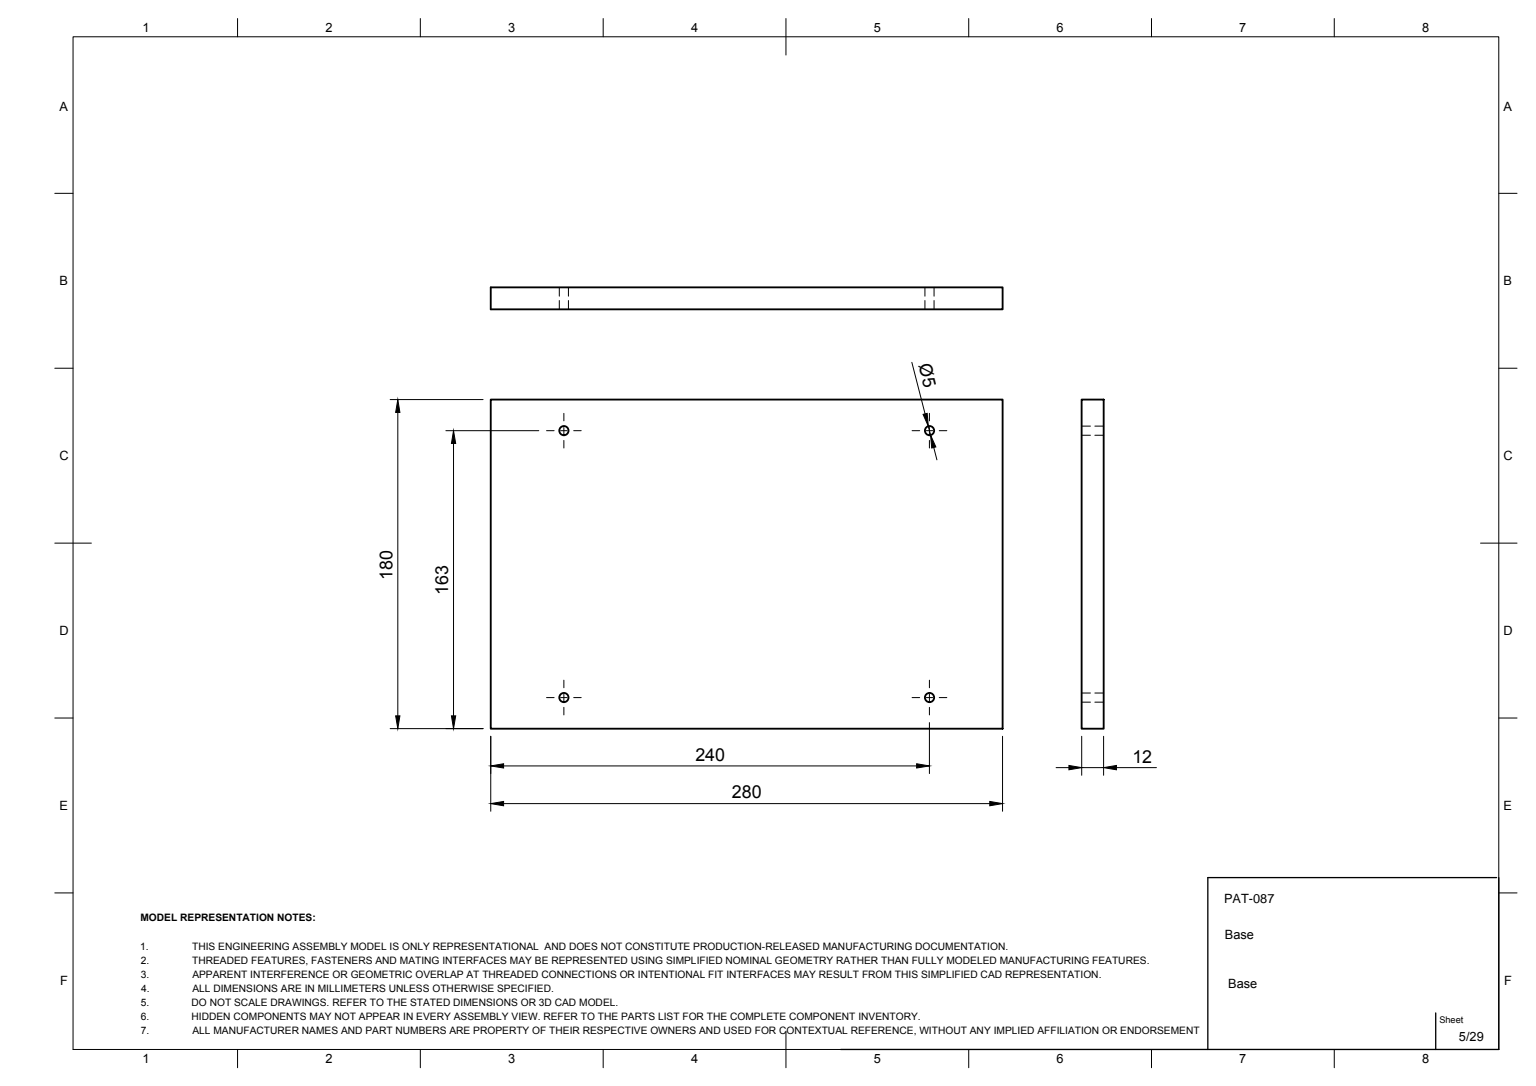
ISO-10303-21;
HEADER;
/* Generated by software containing ST-Developer
 * from STEP Tools, Inc. (www.steptools.com) 
 */

FILE_DESCRIPTION(
/* description */ ('Rigid flange shaft coupling assembly'),
/* implementation_level */ '2;1');

FILE_NAME(
/* name */ 'Base.step',
/* time_stamp */ '2026-10-27T10:47:16-07:00',
/* author */ (''),
/* organization */ (''),
/* preprocessor_version */ 'ST-DEVELOPER v20.2',
/* originating_system */ 'Autodesk Translation Framework v15.17.0.0',
/* authorisation */ '');

FILE_SCHEMA (('AUTOMOTIVE_DESIGN { 1 0 10303 214 3 1 1 }'));
ENDSEC;

DATA;
#10=MECHANICAL_DESIGN_GEOMETRIC_PRESENTATION_REPRESENTATION('',(#398),#9141);
#342=SHAPE_REPRESENTATION_RELATIONSHIP('SRR','None',#9276,#370);
#370=ADVANCED_BREP_SHAPE_REPRESENTATION('',(#427),#9111);
#398=STYLED_ITEM('',(#9479),#427);
#427=MANIFOLD_SOLID_BREP('Body1',#4752);
#453=FACE_BOUND('',#1025,.T.);
#454=FACE_BOUND('',#1026,.T.);
#455=FACE_BOUND('',#1027,.T.);
#456=FACE_BOUND('',#1028,.T.);
#457=FACE_BOUND('',#1030,.T.);
#458=FACE_BOUND('',#1031,.T.);
#459=FACE_BOUND('',#1032,.T.);
#460=FACE_BOUND('',#1033,.T.);
#570=PLANE('',#5108);
#571=PLANE('',#5109);
#572=PLANE('',#5110);
#573=PLANE('',#5111);
#574=PLANE('',#5112);
#575=PLANE('',#5113);
#744=FACE_OUTER_BOUND('',#1016,.T.);
#745=FACE_OUTER_BOUND('',#1017,.T.);
#746=FACE_OUTER_BOUND('',#1018,.T.);
#747=FACE_OUTER_BOUND('',#1019,.T.);
#748=FACE_OUTER_BOUND('',#1020,.T.);
#749=FACE_OUTER_BOUND('',#1021,.T.);
#750=FACE_OUTER_BOUND('',#1022,.T.);
#751=FACE_OUTER_BOUND('',#1023,.T.);
#752=FACE_OUTER_BOUND('',#1024,.T.);
#753=FACE_OUTER_BOUND('',#1029,.T.);
#1016=EDGE_LOOP('',(#3243,#3244,#3245,#3246));
#1017=EDGE_LOOP('',(#3247,#3248,#3249,#3250));
#1018=EDGE_LOOP('',(#3251,#3252,#3253,#3254));
#1019=EDGE_LOOP('',(#3255,#3256,#3257,#3258));
#1020=EDGE_LOOP('',(#3259,#3260,#3261,#3262));
#1021=EDGE_LOOP('',(#3263,#3264,#3265,#3266));
#1022=EDGE_LOOP('',(#3267,#3268,#3269,#3270));
#1023=EDGE_LOOP('',(#3271,#3272,#3273,#3274));
#1024=EDGE_LOOP('',(#3275,#3276,#3277,#3278));
#1025=EDGE_LOOP('',(#3279));
#1026=EDGE_LOOP('',(#3280));
#1027=EDGE_LOOP('',(#3281));
#1028=EDGE_LOOP('',(#3282));
#1029=EDGE_LOOP('',(#3283,#3284,#3285,#3286));
#1030=EDGE_LOOP('',(#3287));
#1031=EDGE_LOOP('',(#3288));
#1032=EDGE_LOOP('',(#3289));
#1033=EDGE_LOOP('',(#3290));
#1405=LINE('',#7092,#1750);
#1406=LINE('',#7098,#1751);
#1407=LINE('',#7104,#1752);
#1408=LINE('',#7110,#1753);
#1409=LINE('',#7115,#1754);
#1410=LINE('',#7117,#1755);
#1411=LINE('',#7119,#1756);
#1412=LINE('',#7120,#1757);
#1413=LINE('',#7123,#1758);
#1414=LINE('',#7125,#1759);
#1415=LINE('',#7126,#1760);
#1416=LINE('',#7129,#1761);
#1417=LINE('',#7131,#1762);
#1418=LINE('',#7132,#1763);
#1419=LINE('',#7134,#1764);
#1420=LINE('',#7135,#1765);
#1750=VECTOR('',#5652,0.25);
#1751=VECTOR('',#5659,0.25);
#1752=VECTOR('',#5666,0.25);
#1753=VECTOR('',#5673,0.25);
#1754=VECTOR('',#5678,1.);
#1755=VECTOR('',#5679,1.);
#1756=VECTOR('',#5680,1.);
#1757=VECTOR('',#5681,1.);
#1758=VECTOR('',#5684,1.);
#1759=VECTOR('',#5685,1.);
#1760=VECTOR('',#5686,1.);
#1761=VECTOR('',#5689,1.);
#1762=VECTOR('',#5690,1.);
#1763=VECTOR('',#5691,1.);
#1764=VECTOR('',#5694,1.);
#1765=VECTOR('',#5695,1.);
#2095=CIRCLE('',#5097,0.25);
#2096=CIRCLE('',#5098,0.25);
#2097=CIRCLE('',#5100,0.25);
#2098=CIRCLE('',#5101,0.25);
#2099=CIRCLE('',#5103,0.25);
#2100=CIRCLE('',#5104,0.25);
#2101=CIRCLE('',#5106,0.25);
#2102=CIRCLE('',#5107,0.25);
#2276=VERTEX_POINT('',#7089);
#2277=VERTEX_POINT('',#7091);
#2278=VERTEX_POINT('',#7095);
#2279=VERTEX_POINT('',#7097);
#2280=VERTEX_POINT('',#7101);
#2281=VERTEX_POINT('',#7103);
#2282=VERTEX_POINT('',#7107);
#2283=VERTEX_POINT('',#7109);
#2284=VERTEX_POINT('',#7113);
#2285=VERTEX_POINT('',#7114);
#2286=VERTEX_POINT('',#7116);
#2287=VERTEX_POINT('',#7118);
#2288=VERTEX_POINT('',#7122);
#2289=VERTEX_POINT('',#7124);
#2290=VERTEX_POINT('',#7128);
#2291=VERTEX_POINT('',#7130);
#2665=EDGE_CURVE('',#2276,#2276,#2095,.T.);
#2666=EDGE_CURVE('',#2276,#2277,#1405,.T.);
#2667=EDGE_CURVE('',#2277,#2277,#2096,.T.);
#2668=EDGE_CURVE('',#2278,#2278,#2097,.T.);
#2669=EDGE_CURVE('',#2278,#2279,#1406,.T.);
#2670=EDGE_CURVE('',#2279,#2279,#2098,.T.);
#2671=EDGE_CURVE('',#2280,#2280,#2099,.T.);
#2672=EDGE_CURVE('',#2280,#2281,#1407,.T.);
#2673=EDGE_CURVE('',#2281,#2281,#2100,.T.);
#2674=EDGE_CURVE('',#2282,#2282,#2101,.T.);
#2675=EDGE_CURVE('',#2282,#2283,#1408,.T.);
#2676=EDGE_CURVE('',#2283,#2283,#2102,.T.);
#2677=EDGE_CURVE('',#2284,#2285,#1409,.T.);
#2678=EDGE_CURVE('',#2285,#2286,#1410,.T.);
#2679=EDGE_CURVE('',#2287,#2286,#1411,.T.);
#2680=EDGE_CURVE('',#2284,#2287,#1412,.T.);
#2681=EDGE_CURVE('',#2288,#2284,#1413,.T.);
#2682=EDGE_CURVE('',#2289,#2287,#1414,.T.);
#2683=EDGE_CURVE('',#2288,#2289,#1415,.T.);
#2684=EDGE_CURVE('',#2290,#2288,#1416,.T.);
#2685=EDGE_CURVE('',#2291,#2289,#1417,.T.);
#2686=EDGE_CURVE('',#2290,#2291,#1418,.T.);
#2687=EDGE_CURVE('',#2285,#2290,#1419,.T.);
#2688=EDGE_CURVE('',#2286,#2291,#1420,.T.);
#3243=ORIENTED_EDGE('',*,*,#2665,.F.);
#3244=ORIENTED_EDGE('',*,*,#2666,.T.);
#3245=ORIENTED_EDGE('',*,*,#2667,.F.);
#3246=ORIENTED_EDGE('',*,*,#2666,.F.);
#3247=ORIENTED_EDGE('',*,*,#2668,.F.);
#3248=ORIENTED_EDGE('',*,*,#2669,.T.);
#3249=ORIENTED_EDGE('',*,*,#2670,.F.);
#3250=ORIENTED_EDGE('',*,*,#2669,.F.);
#3251=ORIENTED_EDGE('',*,*,#2671,.F.);
#3252=ORIENTED_EDGE('',*,*,#2672,.T.);
#3253=ORIENTED_EDGE('',*,*,#2673,.F.);
#3254=ORIENTED_EDGE('',*,*,#2672,.F.);
#3255=ORIENTED_EDGE('',*,*,#2674,.F.);
#3256=ORIENTED_EDGE('',*,*,#2675,.T.);
#3257=ORIENTED_EDGE('',*,*,#2676,.F.);
#3258=ORIENTED_EDGE('',*,*,#2675,.F.);
#3259=ORIENTED_EDGE('',*,*,#2677,.T.);
#3260=ORIENTED_EDGE('',*,*,#2678,.T.);
#3261=ORIENTED_EDGE('',*,*,#2679,.F.);
#3262=ORIENTED_EDGE('',*,*,#2680,.F.);
#3263=ORIENTED_EDGE('',*,*,#2681,.T.);
#3264=ORIENTED_EDGE('',*,*,#2680,.T.);
#3265=ORIENTED_EDGE('',*,*,#2682,.F.);
#3266=ORIENTED_EDGE('',*,*,#2683,.F.);
#3267=ORIENTED_EDGE('',*,*,#2684,.T.);
#3268=ORIENTED_EDGE('',*,*,#2683,.T.);
#3269=ORIENTED_EDGE('',*,*,#2685,.F.);
#3270=ORIENTED_EDGE('',*,*,#2686,.F.);
#3271=ORIENTED_EDGE('',*,*,#2687,.T.);
#3272=ORIENTED_EDGE('',*,*,#2686,.T.);
#3273=ORIENTED_EDGE('',*,*,#2688,.F.);
#3274=ORIENTED_EDGE('',*,*,#2678,.F.);
#3275=ORIENTED_EDGE('',*,*,#2688,.T.);
#3276=ORIENTED_EDGE('',*,*,#2685,.T.);
#3277=ORIENTED_EDGE('',*,*,#2682,.T.);
#3278=ORIENTED_EDGE('',*,*,#2679,.T.);
#3279=ORIENTED_EDGE('',*,*,#2667,.T.);
#3280=ORIENTED_EDGE('',*,*,#2670,.T.);
#3281=ORIENTED_EDGE('',*,*,#2673,.T.);
#3282=ORIENTED_EDGE('',*,*,#2676,.T.);
#3283=ORIENTED_EDGE('',*,*,#2687,.F.);
#3284=ORIENTED_EDGE('',*,*,#2677,.F.);
#3285=ORIENTED_EDGE('',*,*,#2681,.F.);
#3286=ORIENTED_EDGE('',*,*,#2684,.F.);
#3287=ORIENTED_EDGE('',*,*,#2665,.T.);
#3288=ORIENTED_EDGE('',*,*,#2668,.T.);
#3289=ORIENTED_EDGE('',*,*,#2671,.T.);
#3290=ORIENTED_EDGE('',*,*,#2674,.T.);
#4399=CYLINDRICAL_SURFACE('',#5096,0.25);
#4400=CYLINDRICAL_SURFACE('',#5099,0.25);
#4401=CYLINDRICAL_SURFACE('',#5102,0.25);
#4402=CYLINDRICAL_SURFACE('',#5105,0.25);
#4480=ADVANCED_FACE('',(#744),#4399,.F.);
#4481=ADVANCED_FACE('',(#745),#4400,.F.);
#4482=ADVANCED_FACE('',(#746),#4401,.F.);
#4483=ADVANCED_FACE('',(#747),#4402,.F.);
#4484=ADVANCED_FACE('',(#748),#570,.T.);
#4485=ADVANCED_FACE('',(#749),#571,.T.);
#4486=ADVANCED_FACE('',(#750),#572,.T.);
#4487=ADVANCED_FACE('',(#751),#573,.T.);
#4488=ADVANCED_FACE('',(#752,#453,#454,#455,#456),#574,.T.);
#4489=ADVANCED_FACE('',(#753,#457,#458,#459,#460),#575,.F.);
#4752=CLOSED_SHELL('',(#4480,#4481,#4482,#4483,#4484,#4485,#4486,#4487,
#4488,#4489));
#5095=AXIS2_PLACEMENT_3D('',#7087,#5646,#5647);
#5096=AXIS2_PLACEMENT_3D('',#7088,#5648,#5649);
#5097=AXIS2_PLACEMENT_3D('',#7090,#5650,#5651);
#5098=AXIS2_PLACEMENT_3D('',#7093,#5653,#5654);
#5099=AXIS2_PLACEMENT_3D('',#7094,#5655,#5656);
#5100=AXIS2_PLACEMENT_3D('',#7096,#5657,#5658);
#5101=AXIS2_PLACEMENT_3D('',#7099,#5660,#5661);
#5102=AXIS2_PLACEMENT_3D('',#7100,#5662,#5663);
#5103=AXIS2_PLACEMENT_3D('',#7102,#5664,#5665);
#5104=AXIS2_PLACEMENT_3D('',#7105,#5667,#5668);
#5105=AXIS2_PLACEMENT_3D('',#7106,#5669,#5670);
#5106=AXIS2_PLACEMENT_3D('',#7108,#5671,#5672);
#5107=AXIS2_PLACEMENT_3D('',#7111,#5674,#5675);
#5108=AXIS2_PLACEMENT_3D('',#7112,#5676,#5677);
#5109=AXIS2_PLACEMENT_3D('',#7121,#5682,#5683);
#5110=AXIS2_PLACEMENT_3D('',#7127,#5687,#5688);
#5111=AXIS2_PLACEMENT_3D('',#7133,#5692,#5693);
#5112=AXIS2_PLACEMENT_3D('',#7136,#5696,#5697);
#5113=AXIS2_PLACEMENT_3D('',#7137,#5698,#5699);
#5646=DIRECTION('axis',(0.,0.,1.));
#5647=DIRECTION('refdir',(1.,0.,0.));
#5648=DIRECTION('center_axis',(0.,0.,1.));
#5649=DIRECTION('ref_axis',(1.,0.,0.));
#5650=DIRECTION('center_axis',(0.,0.,1.));
#5651=DIRECTION('ref_axis',(1.,0.,0.));
#5652=DIRECTION('',(0.,0.,1.));
#5653=DIRECTION('center_axis',(0.,0.,-1.));
#5654=DIRECTION('ref_axis',(1.,0.,0.));
#5655=DIRECTION('center_axis',(0.,0.,1.));
#5656=DIRECTION('ref_axis',(1.,0.,0.));
#5657=DIRECTION('center_axis',(0.,0.,1.));
#5658=DIRECTION('ref_axis',(1.,0.,0.));
#5659=DIRECTION('',(0.,0.,1.));
#5660=DIRECTION('center_axis',(0.,0.,-1.));
#5661=DIRECTION('ref_axis',(1.,0.,0.));
#5662=DIRECTION('center_axis',(0.,0.,1.));
#5663=DIRECTION('ref_axis',(1.,0.,0.));
#5664=DIRECTION('center_axis',(0.,0.,1.));
#5665=DIRECTION('ref_axis',(1.,0.,0.));
#5666=DIRECTION('',(0.,0.,1.));
#5667=DIRECTION('center_axis',(0.,0.,-1.));
#5668=DIRECTION('ref_axis',(1.,0.,0.));
#5669=DIRECTION('center_axis',(0.,0.,1.));
#5670=DIRECTION('ref_axis',(1.,0.,0.));
#5671=DIRECTION('center_axis',(0.,0.,1.));
#5672=DIRECTION('ref_axis',(1.,0.,0.));
#5673=DIRECTION('',(0.,0.,1.));
#5674=DIRECTION('center_axis',(0.,0.,-1.));
#5675=DIRECTION('ref_axis',(1.,0.,0.));
#5676=DIRECTION('center_axis',(0.,1.,0.));
#5677=DIRECTION('ref_axis',(-1.,0.,0.));
#5678=DIRECTION('',(-1.,0.,0.));
#5679=DIRECTION('',(0.,0.,1.));
#5680=DIRECTION('',(-1.,0.,0.));
#5681=DIRECTION('',(0.,0.,1.));
#5682=DIRECTION('center_axis',(1.,0.,0.));
#5683=DIRECTION('ref_axis',(0.,1.,0.));
#5684=DIRECTION('',(0.,1.,0.));
#5685=DIRECTION('',(0.,1.,0.));
#5686=DIRECTION('',(0.,0.,1.));
#5687=DIRECTION('center_axis',(0.,-1.,0.));
#5688=DIRECTION('ref_axis',(1.,0.,0.));
#5689=DIRECTION('',(1.,0.,0.));
#5690=DIRECTION('',(1.,0.,0.));
#5691=DIRECTION('',(0.,0.,1.));
#5692=DIRECTION('center_axis',(-1.,0.,0.));
#5693=DIRECTION('ref_axis',(0.,-1.,0.));
#5694=DIRECTION('',(0.,-1.,0.));
#5695=DIRECTION('',(0.,-1.,0.));
#5696=DIRECTION('center_axis',(0.,0.,1.));
#5697=DIRECTION('ref_axis',(1.,0.,0.));
#5698=DIRECTION('center_axis',(0.,0.,1.));
#5699=DIRECTION('ref_axis',(1.,0.,0.));
#7087=CARTESIAN_POINT('',(0.,0.,0.));
#7088=CARTESIAN_POINT('Origin',(7.3,0.,-0.1));
#7089=CARTESIAN_POINT('',(7.05,-3.06161699786838E-17,0.));
#7090=CARTESIAN_POINT('Origin',(7.3,0.,0.));
#7091=CARTESIAN_POINT('',(7.05,3.06161699786838E-17,1.2));
#7092=CARTESIAN_POINT('',(7.05,-3.06161699786838E-17,-0.1));
#7093=CARTESIAN_POINT('Origin',(7.3,0.,1.2));
#7094=CARTESIAN_POINT('Origin',(-7.3,20.,-0.1));
#7095=CARTESIAN_POINT('',(-7.55,20.,0.));
#7096=CARTESIAN_POINT('Origin',(-7.3,20.,0.));
#7097=CARTESIAN_POINT('',(-7.55,20.,1.2));
#7098=CARTESIAN_POINT('',(-7.55,20.,-0.1));
#7099=CARTESIAN_POINT('Origin',(-7.3,20.,1.2));
#7100=CARTESIAN_POINT('Origin',(-7.3,0.,-0.1));
#7101=CARTESIAN_POINT('',(-7.55,-3.06161699786838E-17,0.));
#7102=CARTESIAN_POINT('Origin',(-7.3,0.,0.));
#7103=CARTESIAN_POINT('',(-7.55,3.06161699786838E-17,1.2));
#7104=CARTESIAN_POINT('',(-7.55,-3.06161699786838E-17,-0.1));
#7105=CARTESIAN_POINT('Origin',(-7.3,0.,1.2));
#7106=CARTESIAN_POINT('Origin',(7.3,20.,-0.1));
#7107=CARTESIAN_POINT('',(7.05,20.,0.));
#7108=CARTESIAN_POINT('Origin',(7.3,20.,0.));
#7109=CARTESIAN_POINT('',(7.05,20.,1.2));
#7110=CARTESIAN_POINT('',(7.05,20.,-0.1));
#7111=CARTESIAN_POINT('Origin',(7.3,20.,1.2));
#7112=CARTESIAN_POINT('Origin',(9.,24.,0.));
#7113=CARTESIAN_POINT('',(9.,24.,0.));
#7114=CARTESIAN_POINT('',(-9.,24.,0.));
#7115=CARTESIAN_POINT('',(9.,24.,0.));
#7116=CARTESIAN_POINT('',(-9.,24.,1.2));
#7117=CARTESIAN_POINT('',(-9.,24.,0.));
#7118=CARTESIAN_POINT('',(9.,24.,1.2));
#7119=CARTESIAN_POINT('',(9.,24.,1.2));
#7120=CARTESIAN_POINT('',(9.,24.,0.));
#7121=CARTESIAN_POINT('Origin',(9.,-4.,0.));
#7122=CARTESIAN_POINT('',(9.,-4.,0.));
#7123=CARTESIAN_POINT('',(9.,-4.,0.));
#7124=CARTESIAN_POINT('',(9.,-4.,1.2));
#7125=CARTESIAN_POINT('',(9.,-4.,1.2));
#7126=CARTESIAN_POINT('',(9.,-4.,0.));
#7127=CARTESIAN_POINT('Origin',(-9.,-4.,0.));
#7128=CARTESIAN_POINT('',(-9.,-4.,0.));
#7129=CARTESIAN_POINT('',(-9.,-4.,0.));
#7130=CARTESIAN_POINT('',(-9.,-4.,1.2));
#7131=CARTESIAN_POINT('',(-9.,-4.,1.2));
#7132=CARTESIAN_POINT('',(-9.,-4.,0.));
#7133=CARTESIAN_POINT('Origin',(-9.,24.,0.));
#7134=CARTESIAN_POINT('',(-9.,24.,0.));
#7135=CARTESIAN_POINT('',(-9.,24.,1.2));
#7136=CARTESIAN_POINT('Origin',(0.,10.,1.2));
#7137=CARTESIAN_POINT('Origin',(0.,10.,0.));
#9078=UNCERTAINTY_MEASURE_WITH_UNIT(LENGTH_MEASURE(0.001),#9142,
'DISTANCE_ACCURACY_VALUE',
'Maximum model space distance between geometric entities at asserted c
onnectivities');
#9108=UNCERTAINTY_MEASURE_WITH_UNIT(LENGTH_MEASURE(0.001),#9142,
'DISTANCE_ACCURACY_VALUE',
'Maximum model space distance between geometric entities at asserted c
onnectivities');
#9111=(
GEOMETRIC_REPRESENTATION_CONTEXT(3)
GLOBAL_UNCERTAINTY_ASSIGNED_CONTEXT((#9078))
GLOBAL_UNIT_ASSIGNED_CONTEXT((#9142,#9144,#9145))
REPRESENTATION_CONTEXT('','3D')
);
#9141=(
GEOMETRIC_REPRESENTATION_CONTEXT(3)
GLOBAL_UNCERTAINTY_ASSIGNED_CONTEXT((#9108))
GLOBAL_UNIT_ASSIGNED_CONTEXT((#9142,#9144,#9145))
REPRESENTATION_CONTEXT('','3D')
);
#9142=(
LENGTH_UNIT()
NAMED_UNIT(*)
SI_UNIT(.CENTI.,.METRE.)
);
#9144=(
NAMED_UNIT(*)
PLANE_ANGLE_UNIT()
SI_UNIT($,.RADIAN.)
);
#9145=(
NAMED_UNIT(*)
SI_UNIT($,.STERADIAN.)
SOLID_ANGLE_UNIT()
);
#9148=SHAPE_DEFINITION_REPRESENTATION(#9180,#9276);
#9180=PRODUCT_DEFINITION_SHAPE('',$,#9309);
#9276=SHAPE_REPRESENTATION('',(#5095),#9111);
#9306=PRODUCT_DEFINITION_CONTEXT('part definition',#9404,'design');
#9309=PRODUCT_DEFINITION('Base','Base',#9341,#9306);
#9341=PRODUCT_DEFINITION_FORMATION('',$,#9408);
#9404=APPLICATION_CONTEXT(
'Core Data for Automotive Mechanical Design Process');
#9405=PRODUCT_CONTEXT('part definition',#9404,'mechanical');
#9408=PRODUCT('Base','Base','Base',(#9405));
#9473=COLOUR_RGB('Dark Blue',0.08,0.2,0.34);
#9474=FILL_AREA_STYLE_COLOUR('',#9473);
#9475=FILL_AREA_STYLE('',(#9474));
#9476=SURFACE_STYLE_FILL_AREA(#9475);
#9477=SURFACE_SIDE_STYLE('',(#9476));
#9478=SURFACE_STYLE_USAGE(.BOTH.,#9477);
#9479=PRESENTATION_STYLE_ASSIGNMENT((#9478));
ENDSEC;
END-ISO-10303-21;
